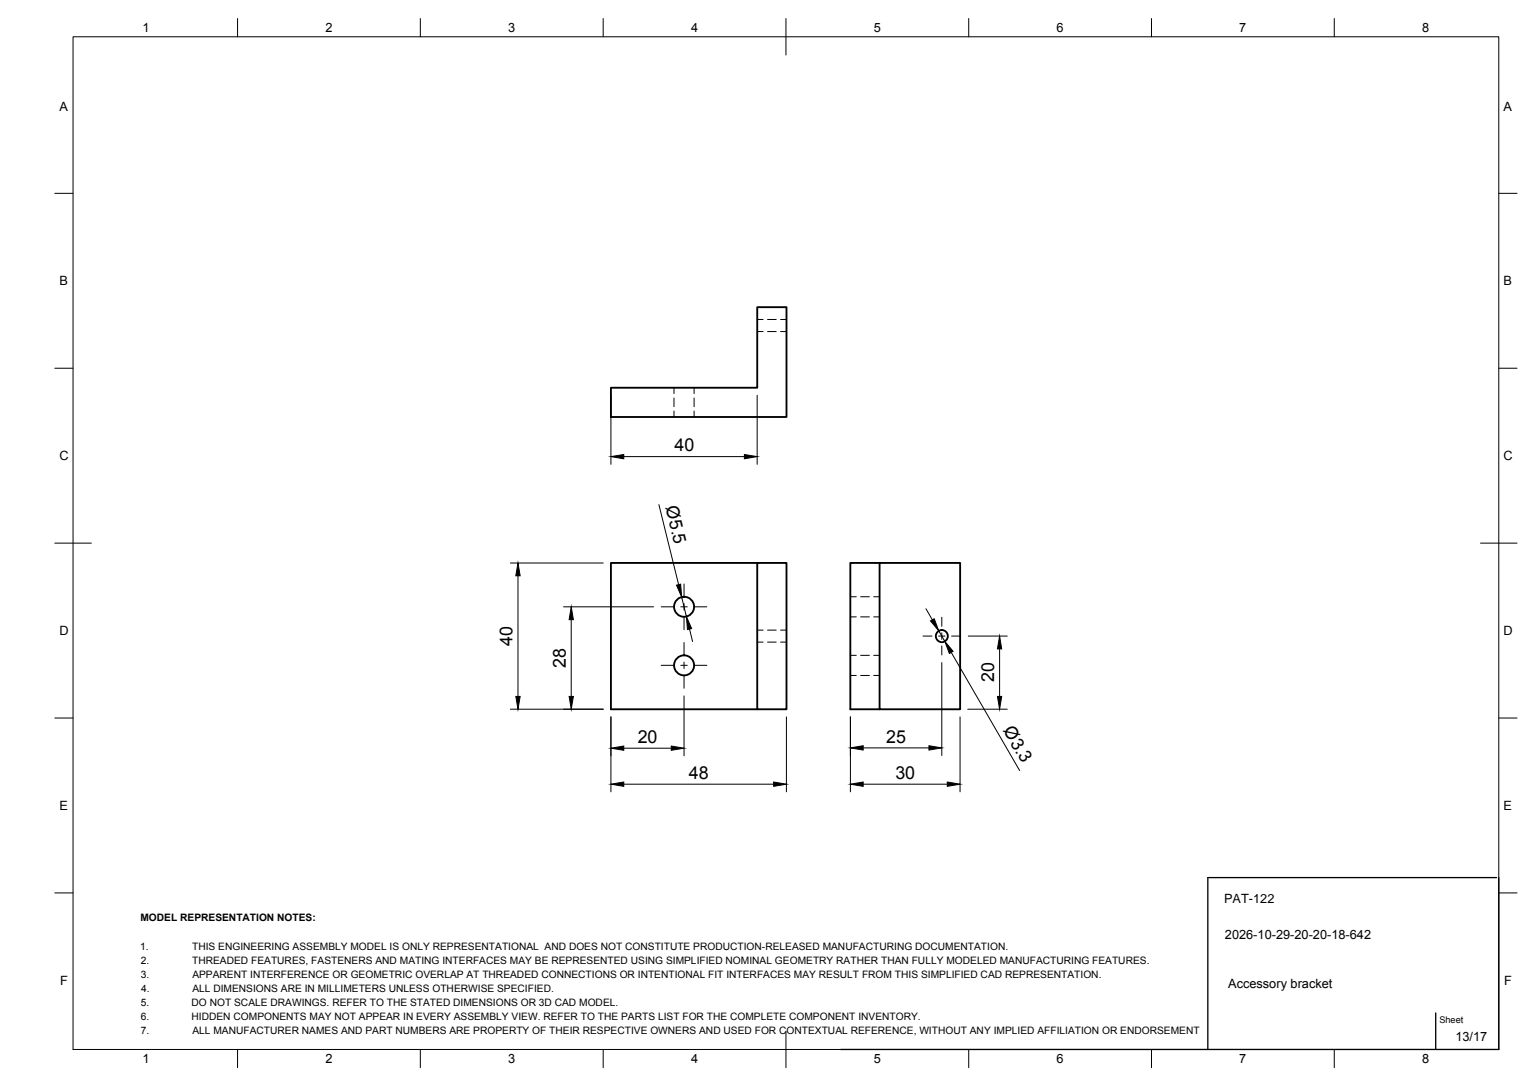
ISO-10303-21;
HEADER;
/* Generated by software containing ST-Developer
 * from STEP Tools, Inc. (www.steptools.com) 
 */

FILE_DESCRIPTION(
/* description */ ('PAT-122'),
/* implementation_level */ '2;1');

FILE_NAME(
/* name */ 'Accessory bracket.step',
/* time_stamp */ '2026-10-29T20:20:12-07:00',
/* author */ (''),
/* organization */ (''),
/* preprocessor_version */ 'ST-DEVELOPER v20.2',
/* originating_system */ 'Autodesk Translation Framework v15.17.0.0',
/* authorisation */ '');

FILE_SCHEMA (('AUTOMOTIVE_DESIGN { 1 0 10303 214 3 1 1 }'));
ENDSEC;

DATA;
#10=MECHANICAL_DESIGN_GEOMETRIC_PRESENTATION_REPRESENTATION('',(#501),#10019);
#457=SHAPE_REPRESENTATION_RELATIONSHIP('SRR','None',#10178,#479);
#479=ADVANCED_BREP_SHAPE_REPRESENTATION('',(#523),#10007);
#501=STYLED_ITEM('',(#10327),#523);
#523=MANIFOLD_SOLID_BREP('Body1',#5623);
#567=FACE_BOUND('',#1225,.T.);
#568=FACE_BOUND('',#1228,.T.);
#569=FACE_BOUND('',#1230,.T.);
#570=FACE_BOUND('',#1231,.T.);
#571=FACE_BOUND('',#1234,.T.);
#572=FACE_BOUND('',#1235,.T.);
#649=PLANE('',#6027);
#650=PLANE('',#6028);
#651=PLANE('',#6029);
#652=PLANE('',#6030);
#653=PLANE('',#6031);
#654=PLANE('',#6032);
#655=PLANE('',#6033);
#656=PLANE('',#6034);
#893=FACE_OUTER_BOUND('',#1221,.T.);
#894=FACE_OUTER_BOUND('',#1222,.T.);
#895=FACE_OUTER_BOUND('',#1223,.T.);
#896=FACE_OUTER_BOUND('',#1224,.T.);
#897=FACE_OUTER_BOUND('',#1226,.T.);
#898=FACE_OUTER_BOUND('',#1227,.T.);
#899=FACE_OUTER_BOUND('',#1229,.T.);
#900=FACE_OUTER_BOUND('',#1232,.T.);
#901=FACE_OUTER_BOUND('',#1233,.T.);
#902=FACE_OUTER_BOUND('',#1236,.T.);
#903=FACE_OUTER_BOUND('',#1237,.T.);
#1221=EDGE_LOOP('',(#4129,#4130,#4131,#4132));
#1222=EDGE_LOOP('',(#4133,#4134,#4135,#4136));
#1223=EDGE_LOOP('',(#4137,#4138,#4139,#4140));
#1224=EDGE_LOOP('',(#4141,#4142,#4143,#4144));
#1225=EDGE_LOOP('',(#4145));
#1226=EDGE_LOOP('',(#4146,#4147,#4148,#4149));
#1227=EDGE_LOOP('',(#4150,#4151,#4152,#4153));
#1228=EDGE_LOOP('',(#4154));
#1229=EDGE_LOOP('',(#4155,#4156,#4157,#4158));
#1230=EDGE_LOOP('',(#4159));
#1231=EDGE_LOOP('',(#4160));
#1232=EDGE_LOOP('',(#4161,#4162,#4163,#4164));
#1233=EDGE_LOOP('',(#4165,#4166,#4167,#4168));
#1234=EDGE_LOOP('',(#4169));
#1235=EDGE_LOOP('',(#4170));
#1236=EDGE_LOOP('',(#4171,#4172,#4173,#4174,#4175,#4176));
#1237=EDGE_LOOP('',(#4177,#4178,#4179,#4180,#4181,#4182));
#1563=LINE('',#8362,#2107);
#1564=LINE('',#8368,#2108);
#1565=LINE('',#8374,#2109);
#1566=LINE('',#8379,#2110);
#1567=LINE('',#8381,#2111);
#1568=LINE('',#8383,#2112);
#1569=LINE('',#8384,#2113);
#1570=LINE('',#8387,#2114);
#1571=LINE('',#8389,#2115);
#1572=LINE('',#8390,#2116);
#1573=LINE('',#8393,#2117);
#1574=LINE('',#8395,#2118);
#1575=LINE('',#8396,#2119);
#1576=LINE('',#8399,#2120);
#1577=LINE('',#8401,#2121);
#1578=LINE('',#8402,#2122);
#1579=LINE('',#8405,#2123);
#1580=LINE('',#8407,#2124);
#1581=LINE('',#8408,#2125);
#1582=LINE('',#8410,#2126);
#1583=LINE('',#8411,#2127);
#2107=VECTOR('',#6778,0.164999999999999);
#2108=VECTOR('',#6785,0.275);
#2109=VECTOR('',#6792,0.275);
#2110=VECTOR('',#6797,1.);
#2111=VECTOR('',#6798,1.);
#2112=VECTOR('',#6799,1.);
#2113=VECTOR('',#6800,1.);
#2114=VECTOR('',#6803,1.);
#2115=VECTOR('',#6804,1.);
#2116=VECTOR('',#6805,1.);
#2117=VECTOR('',#6808,1.);
#2118=VECTOR('',#6809,1.);
#2119=VECTOR('',#6810,1.);
#2120=VECTOR('',#6813,1.);
#2121=VECTOR('',#6814,1.);
#2122=VECTOR('',#6815,1.);
#2123=VECTOR('',#6818,1.);
#2124=VECTOR('',#6819,1.);
#2125=VECTOR('',#6820,1.);
#2126=VECTOR('',#6823,1.);
#2127=VECTOR('',#6824,1.);
#2631=CIRCLE('',#6019,0.164999999999999);
#2632=CIRCLE('',#6020,0.164999999999999);
#2633=CIRCLE('',#6022,0.275);
#2634=CIRCLE('',#6023,0.275);
#2635=CIRCLE('',#6025,0.275);
#2636=CIRCLE('',#6026,0.275);
#2793=VERTEX_POINT('',#8359);
#2794=VERTEX_POINT('',#8361);
#2795=VERTEX_POINT('',#8365);
#2796=VERTEX_POINT('',#8367);
#2797=VERTEX_POINT('',#8371);
#2798=VERTEX_POINT('',#8373);
#2799=VERTEX_POINT('',#8377);
#2800=VERTEX_POINT('',#8378);
#2801=VERTEX_POINT('',#8380);
#2802=VERTEX_POINT('',#8382);
#2803=VERTEX_POINT('',#8386);
#2804=VERTEX_POINT('',#8388);
#2805=VERTEX_POINT('',#8392);
#2806=VERTEX_POINT('',#8394);
#2807=VERTEX_POINT('',#8398);
#2808=VERTEX_POINT('',#8400);
#2809=VERTEX_POINT('',#8404);
#2810=VERTEX_POINT('',#8406);
#3299=EDGE_CURVE('',#2793,#2793,#2631,.T.);
#3300=EDGE_CURVE('',#2793,#2794,#1563,.T.);
#3301=EDGE_CURVE('',#2794,#2794,#2632,.T.);
#3302=EDGE_CURVE('',#2795,#2795,#2633,.T.);
#3303=EDGE_CURVE('',#2795,#2796,#1564,.T.);
#3304=EDGE_CURVE('',#2796,#2796,#2634,.T.);
#3305=EDGE_CURVE('',#2797,#2797,#2635,.T.);
#3306=EDGE_CURVE('',#2797,#2798,#1565,.T.);
#3307=EDGE_CURVE('',#2798,#2798,#2636,.T.);
#3308=EDGE_CURVE('',#2799,#2800,#1566,.T.);
#3309=EDGE_CURVE('',#2800,#2801,#1567,.T.);
#3310=EDGE_CURVE('',#2802,#2801,#1568,.T.);
#3311=EDGE_CURVE('',#2799,#2802,#1569,.T.);
#3312=EDGE_CURVE('',#2803,#2799,#1570,.T.);
#3313=EDGE_CURVE('',#2804,#2802,#1571,.T.);
#3314=EDGE_CURVE('',#2803,#2804,#1572,.T.);
#3315=EDGE_CURVE('',#2805,#2803,#1573,.T.);
#3316=EDGE_CURVE('',#2806,#2804,#1574,.T.);
#3317=EDGE_CURVE('',#2805,#2806,#1575,.T.);
#3318=EDGE_CURVE('',#2807,#2805,#1576,.T.);
#3319=EDGE_CURVE('',#2808,#2806,#1577,.T.);
#3320=EDGE_CURVE('',#2807,#2808,#1578,.T.);
#3321=EDGE_CURVE('',#2809,#2807,#1579,.T.);
#3322=EDGE_CURVE('',#2810,#2808,#1580,.T.);
#3323=EDGE_CURVE('',#2809,#2810,#1581,.T.);
#3324=EDGE_CURVE('',#2800,#2809,#1582,.T.);
#3325=EDGE_CURVE('',#2801,#2810,#1583,.T.);
#4129=ORIENTED_EDGE('',*,*,#3299,.F.);
#4130=ORIENTED_EDGE('',*,*,#3300,.T.);
#4131=ORIENTED_EDGE('',*,*,#3301,.F.);
#4132=ORIENTED_EDGE('',*,*,#3300,.F.);
#4133=ORIENTED_EDGE('',*,*,#3302,.F.);
#4134=ORIENTED_EDGE('',*,*,#3303,.T.);
#4135=ORIENTED_EDGE('',*,*,#3304,.F.);
#4136=ORIENTED_EDGE('',*,*,#3303,.F.);
#4137=ORIENTED_EDGE('',*,*,#3305,.F.);
#4138=ORIENTED_EDGE('',*,*,#3306,.T.);
#4139=ORIENTED_EDGE('',*,*,#3307,.F.);
#4140=ORIENTED_EDGE('',*,*,#3306,.F.);
#4141=ORIENTED_EDGE('',*,*,#3308,.T.);
#4142=ORIENTED_EDGE('',*,*,#3309,.T.);
#4143=ORIENTED_EDGE('',*,*,#3310,.F.);
#4144=ORIENTED_EDGE('',*,*,#3311,.F.);
#4145=ORIENTED_EDGE('',*,*,#3301,.T.);
#4146=ORIENTED_EDGE('',*,*,#3312,.T.);
#4147=ORIENTED_EDGE('',*,*,#3311,.T.);
#4148=ORIENTED_EDGE('',*,*,#3313,.F.);
#4149=ORIENTED_EDGE('',*,*,#3314,.F.);
#4150=ORIENTED_EDGE('',*,*,#3315,.T.);
#4151=ORIENTED_EDGE('',*,*,#3314,.T.);
#4152=ORIENTED_EDGE('',*,*,#3316,.F.);
#4153=ORIENTED_EDGE('',*,*,#3317,.F.);
#4154=ORIENTED_EDGE('',*,*,#3299,.T.);
#4155=ORIENTED_EDGE('',*,*,#3318,.T.);
#4156=ORIENTED_EDGE('',*,*,#3317,.T.);
#4157=ORIENTED_EDGE('',*,*,#3319,.F.);
#4158=ORIENTED_EDGE('',*,*,#3320,.F.);
#4159=ORIENTED_EDGE('',*,*,#3304,.T.);
#4160=ORIENTED_EDGE('',*,*,#3307,.T.);
#4161=ORIENTED_EDGE('',*,*,#3321,.T.);
#4162=ORIENTED_EDGE('',*,*,#3320,.T.);
#4163=ORIENTED_EDGE('',*,*,#3322,.F.);
#4164=ORIENTED_EDGE('',*,*,#3323,.F.);
#4165=ORIENTED_EDGE('',*,*,#3324,.T.);
#4166=ORIENTED_EDGE('',*,*,#3323,.T.);
#4167=ORIENTED_EDGE('',*,*,#3325,.F.);
#4168=ORIENTED_EDGE('',*,*,#3309,.F.);
#4169=ORIENTED_EDGE('',*,*,#3302,.T.);
#4170=ORIENTED_EDGE('',*,*,#3305,.T.);
#4171=ORIENTED_EDGE('',*,*,#3325,.T.);
#4172=ORIENTED_EDGE('',*,*,#3322,.T.);
#4173=ORIENTED_EDGE('',*,*,#3319,.T.);
#4174=ORIENTED_EDGE('',*,*,#3316,.T.);
#4175=ORIENTED_EDGE('',*,*,#3313,.T.);
#4176=ORIENTED_EDGE('',*,*,#3310,.T.);
#4177=ORIENTED_EDGE('',*,*,#3324,.F.);
#4178=ORIENTED_EDGE('',*,*,#3308,.F.);
#4179=ORIENTED_EDGE('',*,*,#3312,.F.);
#4180=ORIENTED_EDGE('',*,*,#3315,.F.);
#4181=ORIENTED_EDGE('',*,*,#3318,.F.);
#4182=ORIENTED_EDGE('',*,*,#3321,.F.);
#5289=CYLINDRICAL_SURFACE('',#6018,0.164999999999999);
#5290=CYLINDRICAL_SURFACE('',#6021,0.275);
#5291=CYLINDRICAL_SURFACE('',#6024,0.275);
#5389=ADVANCED_FACE('',(#893),#5289,.F.);
#5390=ADVANCED_FACE('',(#894),#5290,.F.);
#5391=ADVANCED_FACE('',(#895),#5291,.F.);
#5392=ADVANCED_FACE('',(#896,#567),#649,.T.);
#5393=ADVANCED_FACE('',(#897),#650,.T.);
#5394=ADVANCED_FACE('',(#898,#568),#651,.T.);
#5395=ADVANCED_FACE('',(#899,#569,#570),#652,.T.);
#5396=ADVANCED_FACE('',(#900),#653,.T.);
#5397=ADVANCED_FACE('',(#901,#571,#572),#654,.T.);
#5398=ADVANCED_FACE('',(#902),#655,.T.);
#5399=ADVANCED_FACE('',(#903),#656,.F.);
#5623=CLOSED_SHELL('',(#5389,#5390,#5391,#5392,#5393,#5394,#5395,#5396,
#5397,#5398,#5399));
#6017=AXIS2_PLACEMENT_3D('',#8357,#6772,#6773);
#6018=AXIS2_PLACEMENT_3D('',#8358,#6774,#6775);
#6019=AXIS2_PLACEMENT_3D('',#8360,#6776,#6777);
#6020=AXIS2_PLACEMENT_3D('',#8363,#6779,#6780);
#6021=AXIS2_PLACEMENT_3D('',#8364,#6781,#6782);
#6022=AXIS2_PLACEMENT_3D('',#8366,#6783,#6784);
#6023=AXIS2_PLACEMENT_3D('',#8369,#6786,#6787);
#6024=AXIS2_PLACEMENT_3D('',#8370,#6788,#6789);
#6025=AXIS2_PLACEMENT_3D('',#8372,#6790,#6791);
#6026=AXIS2_PLACEMENT_3D('',#8375,#6793,#6794);
#6027=AXIS2_PLACEMENT_3D('',#8376,#6795,#6796);
#6028=AXIS2_PLACEMENT_3D('',#8385,#6801,#6802);
#6029=AXIS2_PLACEMENT_3D('',#8391,#6806,#6807);
#6030=AXIS2_PLACEMENT_3D('',#8397,#6811,#6812);
#6031=AXIS2_PLACEMENT_3D('',#8403,#6816,#6817);
#6032=AXIS2_PLACEMENT_3D('',#8409,#6821,#6822);
#6033=AXIS2_PLACEMENT_3D('',#8412,#6825,#6826);
#6034=AXIS2_PLACEMENT_3D('',#8413,#6827,#6828);
#6772=DIRECTION('axis',(0.,0.,1.));
#6773=DIRECTION('refdir',(1.,0.,0.));
#6774=DIRECTION('center_axis',(0.,0.,1.));
#6775=DIRECTION('ref_axis',(1.,0.,0.));
#6776=DIRECTION('center_axis',(0.,0.,1.));
#6777=DIRECTION('ref_axis',(1.,0.,0.));
#6778=DIRECTION('',(0.,0.,1.));
#6779=DIRECTION('center_axis',(0.,0.,-1.));
#6780=DIRECTION('ref_axis',(1.,0.,0.));
#6781=DIRECTION('center_axis',(0.,1.,0.));
#6782=DIRECTION('ref_axis',(1.,0.,0.));
#6783=DIRECTION('center_axis',(0.,1.,0.));
#6784=DIRECTION('ref_axis',(1.,0.,0.));
#6785=DIRECTION('',(0.,1.,0.));
#6786=DIRECTION('center_axis',(0.,-1.,0.));
#6787=DIRECTION('ref_axis',(1.,0.,0.));
#6788=DIRECTION('center_axis',(0.,1.,0.));
#6789=DIRECTION('ref_axis',(1.,0.,0.));
#6790=DIRECTION('center_axis',(0.,1.,0.));
#6791=DIRECTION('ref_axis',(1.,0.,0.));
#6792=DIRECTION('',(0.,1.,0.));
#6793=DIRECTION('center_axis',(0.,-1.,0.));
#6794=DIRECTION('ref_axis',(1.,0.,0.));
#6795=DIRECTION('center_axis',(0.,0.,1.));
#6796=DIRECTION('ref_axis',(0.,-1.,0.));
#6797=DIRECTION('',(0.,-1.,0.));
#6798=DIRECTION('',(1.,0.,0.));
#6799=DIRECTION('',(0.,-1.,0.));
#6800=DIRECTION('',(1.,0.,0.));
#6801=DIRECTION('center_axis',(0.,1.,0.));
#6802=DIRECTION('ref_axis',(0.,0.,1.));
#6803=DIRECTION('',(0.,0.,1.));
#6804=DIRECTION('',(0.,0.,1.));
#6805=DIRECTION('',(1.,0.,0.));
#6806=DIRECTION('center_axis',(0.,0.,-1.));
#6807=DIRECTION('ref_axis',(0.,1.,0.));
#6808=DIRECTION('',(0.,1.,0.));
#6809=DIRECTION('',(0.,1.,0.));
#6810=DIRECTION('',(1.,0.,0.));
#6811=DIRECTION('center_axis',(0.,1.,0.));
#6812=DIRECTION('ref_axis',(0.,0.,1.));
#6813=DIRECTION('',(0.,0.,1.));
#6814=DIRECTION('',(0.,0.,1.));
#6815=DIRECTION('',(1.,0.,0.));
#6816=DIRECTION('center_axis',(0.,0.,-1.));
#6817=DIRECTION('ref_axis',(0.,1.,0.));
#6818=DIRECTION('',(0.,1.,0.));
#6819=DIRECTION('',(0.,1.,0.));
#6820=DIRECTION('',(1.,0.,0.));
#6821=DIRECTION('center_axis',(0.,-1.,0.));
#6822=DIRECTION('ref_axis',(0.,0.,-1.));
#6823=DIRECTION('',(0.,0.,-1.));
#6824=DIRECTION('',(0.,0.,-1.));
#6825=DIRECTION('center_axis',(1.,0.,0.));
#6826=DIRECTION('ref_axis',(0.,0.,-1.));
#6827=DIRECTION('center_axis',(1.,0.,0.));
#6828=DIRECTION('ref_axis',(0.,0.,-1.));
#8357=CARTESIAN_POINT('',(0.,0.,0.));
#8358=CARTESIAN_POINT('Origin',(-10.,22.5,38.9));
#8359=CARTESIAN_POINT('',(-10.165,22.5,39.));
#8360=CARTESIAN_POINT('Origin',(-10.,22.5,39.));
#8361=CARTESIAN_POINT('',(-10.165,22.5,39.8));
#8362=CARTESIAN_POINT('',(-10.165,22.5,38.9));
#8363=CARTESIAN_POINT('Origin',(-10.,22.5,39.8));
#8364=CARTESIAN_POINT('Origin',(-10.8,19.9,37.));
#8365=CARTESIAN_POINT('',(-11.075,20.,37.));
#8366=CARTESIAN_POINT('Origin',(-10.8,20.,37.));
#8367=CARTESIAN_POINT('',(-11.075,20.8,37.));
#8368=CARTESIAN_POINT('',(-11.075,19.9,37.));
#8369=CARTESIAN_POINT('Origin',(-10.8,20.8,37.));
#8370=CARTESIAN_POINT('Origin',(-9.2,19.9,37.));
#8371=CARTESIAN_POINT('',(-9.475,20.,37.));
#8372=CARTESIAN_POINT('Origin',(-9.2,20.,37.));
#8373=CARTESIAN_POINT('',(-9.475,20.8,37.));
#8374=CARTESIAN_POINT('',(-9.475,19.9,37.));
#8375=CARTESIAN_POINT('Origin',(-9.2,20.8,37.));
#8376=CARTESIAN_POINT('Origin',(-12.,23.,39.8));
#8377=CARTESIAN_POINT('',(-12.,23.,39.8));
#8378=CARTESIAN_POINT('',(-12.,20.,39.8));
#8379=CARTESIAN_POINT('',(-12.,23.,39.8));
#8380=CARTESIAN_POINT('',(-8.,20.,39.8));
#8381=CARTESIAN_POINT('',(-12.,20.,39.8));
#8382=CARTESIAN_POINT('',(-8.,23.,39.8));
#8383=CARTESIAN_POINT('',(-8.,23.,39.8));
#8384=CARTESIAN_POINT('',(-12.,23.,39.8));
#8385=CARTESIAN_POINT('Origin',(-12.,23.,39.));
#8386=CARTESIAN_POINT('',(-12.,23.,39.));
#8387=CARTESIAN_POINT('',(-12.,23.,39.));
#8388=CARTESIAN_POINT('',(-8.,23.,39.));
#8389=CARTESIAN_POINT('',(-8.,23.,39.));
#8390=CARTESIAN_POINT('',(-12.,23.,39.));
#8391=CARTESIAN_POINT('Origin',(-12.,20.8,39.));
#8392=CARTESIAN_POINT('',(-12.,20.8,39.));
#8393=CARTESIAN_POINT('',(-12.,20.8,39.));
#8394=CARTESIAN_POINT('',(-8.,20.8,39.));
#8395=CARTESIAN_POINT('',(-8.,20.8,39.));
#8396=CARTESIAN_POINT('',(-12.,20.8,39.));
#8397=CARTESIAN_POINT('Origin',(-12.,20.8,35.));
#8398=CARTESIAN_POINT('',(-12.,20.8,35.));
#8399=CARTESIAN_POINT('',(-12.,20.8,35.));
#8400=CARTESIAN_POINT('',(-8.,20.8,35.));
#8401=CARTESIAN_POINT('',(-8.,20.8,35.));
#8402=CARTESIAN_POINT('',(-12.,20.8,35.));
#8403=CARTESIAN_POINT('Origin',(-12.,20.,35.));
#8404=CARTESIAN_POINT('',(-12.,20.,35.));
#8405=CARTESIAN_POINT('',(-12.,20.,35.));
#8406=CARTESIAN_POINT('',(-8.,20.,35.));
#8407=CARTESIAN_POINT('',(-8.,20.,35.));
#8408=CARTESIAN_POINT('',(-12.,20.,35.));
#8409=CARTESIAN_POINT('Origin',(-12.,20.,39.8));
#8410=CARTESIAN_POINT('',(-12.,20.,39.8));
#8411=CARTESIAN_POINT('',(-8.,20.,39.8));
#8412=CARTESIAN_POINT('Origin',(-8.,21.5,37.4));
#8413=CARTESIAN_POINT('Origin',(-12.,21.5,37.4));
#9983=UNCERTAINTY_MEASURE_WITH_UNIT(LENGTH_MEASURE(0.001),#10020,
'DISTANCE_ACCURACY_VALUE',
'Maximum model space distance between geometric entities at asserted c
onnectivities');
#9995=UNCERTAINTY_MEASURE_WITH_UNIT(LENGTH_MEASURE(0.001),#10020,
'DISTANCE_ACCURACY_VALUE',
'Maximum model space distance between geometric entities at asserted c
onnectivities');
#10007=(
GEOMETRIC_REPRESENTATION_CONTEXT(3)
GLOBAL_UNCERTAINTY_ASSIGNED_CONTEXT((#9983))
GLOBAL_UNIT_ASSIGNED_CONTEXT((#10020,#10022,#10023))
REPRESENTATION_CONTEXT('','3D')
);
#10019=(
GEOMETRIC_REPRESENTATION_CONTEXT(3)
GLOBAL_UNCERTAINTY_ASSIGNED_CONTEXT((#9995))
GLOBAL_UNIT_ASSIGNED_CONTEXT((#10020,#10022,#10023))
REPRESENTATION_CONTEXT('','3D')
);
#10020=(
LENGTH_UNIT()
NAMED_UNIT(*)
SI_UNIT(.CENTI.,.METRE.)
);
#10022=(
NAMED_UNIT(*)
PLANE_ANGLE_UNIT()
SI_UNIT($,.RADIAN.)
);
#10023=(
NAMED_UNIT(*)
SI_UNIT($,.STERADIAN.)
SOLID_ANGLE_UNIT()
);
#10035=SHAPE_DEFINITION_REPRESENTATION(#10058,#10178);
#10058=PRODUCT_DEFINITION_SHAPE('',$,#10202);
#10178=SHAPE_REPRESENTATION('',(#6017),#10007);
#10190=PRODUCT_DEFINITION_CONTEXT('part definition',#10261,'design');
#10202=PRODUCT_DEFINITION('Accessory bracket',
'Accessory bracket',#10225,#10190);
#10225=PRODUCT_DEFINITION_FORMATION('',$,#10274);
#10261=APPLICATION_CONTEXT(
'Core Data for Automotive Mechanical Design Process');
#10262=PRODUCT_CONTEXT('part definition',#10261,'mechanical');
#10274=PRODUCT('Accessory bracket','Accessory bracket',
'Accessory bracket',(#10262));
#10321=COLOUR_RGB('Dark Blue',0.08,0.2,0.34);
#10322=FILL_AREA_STYLE_COLOUR('',#10321);
#10323=FILL_AREA_STYLE('',(#10322));
#10324=SURFACE_STYLE_FILL_AREA(#10323);
#10325=SURFACE_SIDE_STYLE('',(#10324));
#10326=SURFACE_STYLE_USAGE(.BOTH.,#10325);
#10327=PRESENTATION_STYLE_ASSIGNMENT((#10326));
ENDSEC;
END-ISO-10303-21;
